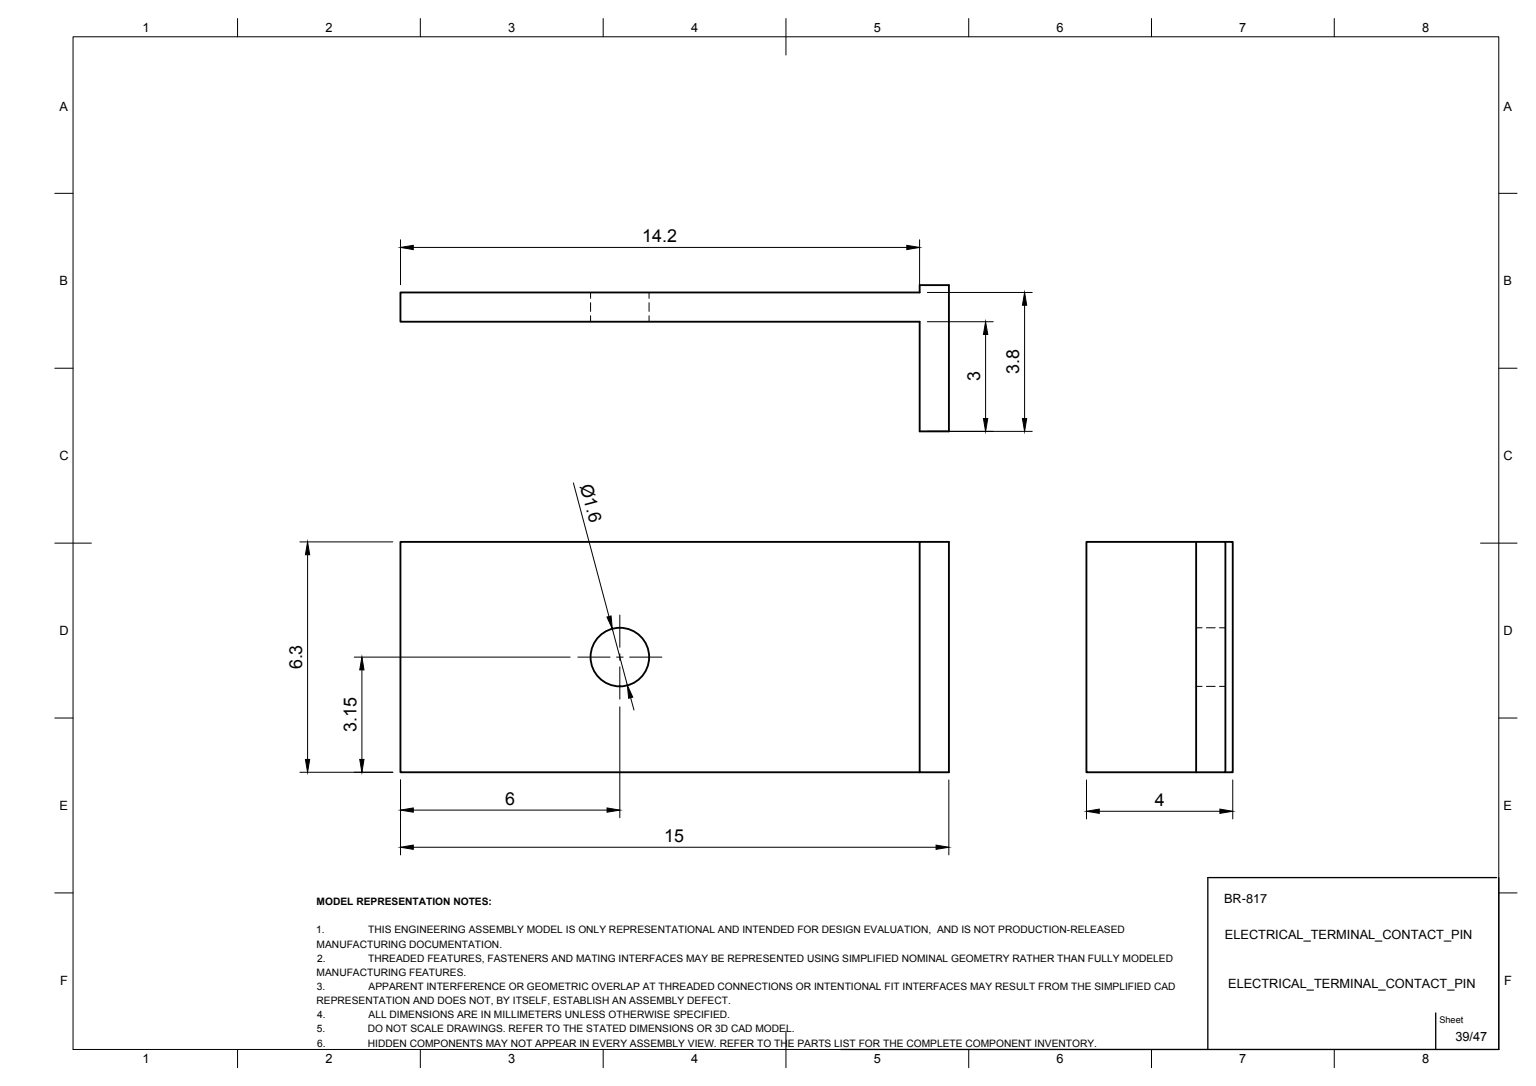
ISO-10303-21;
HEADER;
FILE_DESCRIPTION((''),'2;1');
FILE_NAME('ELECTRICAL_TERMINAL_CONTACT_PIN.step','2026-10-01T22:07:29-07:00',(''),(''),'','','');
FILE_SCHEMA (('AUTOMOTIVE_DESIGN { 1 0 10303 214 3 1 1 }'));
ENDSEC;
DATA;
#10=MECHANICAL_DESIGN_GEOMETRIC_PRESENTATION_REPRESENTATION('',(#570),#15484);
#499=SHAPE_REPRESENTATION_RELATIONSHIP('SRR','None',#15650,#534) ;
#534=ADVANCED_BREP_SHAPE_REPRESENTATION('',(#611),#15474) ;
#570=STYLED_ITEM('',(#15834),#611) ;
#611=MANIFOLD_SOLID_BREP('ELECTRICAL_TERMINAL_CONTACT_PIN',#8281) ;
#793=CYLINDRICAL_SURFACE('',#9781,0.08) ;
#876=FACE_BOUND('',#2357,.T.) ;
#877=FACE_BOUND('',#2360,.T.) ;
#1325=CIRCLE('',#9782,0.08) ;
#1326=CIRCLE('',#9783,0.08) ;
#1789=FACE_OUTER_BOUND('',#2355,.T.) ;
#1790=FACE_OUTER_BOUND('',#2356,.T.) ;
#1791=FACE_OUTER_BOUND('',#2358,.T.) ;
#1792=FACE_OUTER_BOUND('',#2359,.T.) ;
#1793=FACE_OUTER_BOUND('',#2361,.T.) ;
#1794=FACE_OUTER_BOUND('',#2362,.T.) ;
#1795=FACE_OUTER_BOUND('',#2363,.T.) ;
#1796=FACE_OUTER_BOUND('',#2364,.T.) ;
#1797=FACE_OUTER_BOUND('',#2365,.T.) ;
#1798=FACE_OUTER_BOUND('',#2366,.T.) ;
#1799=FACE_OUTER_BOUND('',#2367,.T.) ;
#2355=EDGE_LOOP('',(#7269,#7270,#7271,#7272)) ;
#2356=EDGE_LOOP('',(#7273,#7274,#7275,#7276)) ;
#2357=EDGE_LOOP('',(#7277)) ;
#2358=EDGE_LOOP('',(#7278,#7279,#7280,#7281)) ;
#2359=EDGE_LOOP('',(#7282,#7283,#7284,#7285)) ;
#2360=EDGE_LOOP('',(#7286)) ;
#2361=EDGE_LOOP('',(#7287,#7288,#7289,#7290)) ;
#2362=EDGE_LOOP('',(#7291,#7292,#7293,#7294)) ;
#2363=EDGE_LOOP('',(#7295,#7296,#7297,#7298)) ;
#2364=EDGE_LOOP('',(#7299,#7300,#7301,#7302,#7303,#7304,#7305,#7306)) ;
#2365=EDGE_LOOP('',(#7307,#7308,#7309,#7310)) ;
#2366=EDGE_LOOP('',(#7311,#7312,#7313,#7314,#7315,#7316,#7317,#7318)) ;
#2367=EDGE_LOOP('',(#7319,#7320,#7321,#7322)) ;
#2820=LINE('',#15076,#3294) ;
#2821=LINE('',#15081,#3295) ;
#2822=LINE('',#15083,#3296) ;
#2823=LINE('',#15085,#3297) ;
#2824=LINE('',#15086,#3298) ;
#2825=LINE('',#15090,#3299) ;
#2826=LINE('',#15091,#3300) ;
#2827=LINE('',#15092,#3301) ;
#2828=LINE('',#15096,#3302) ;
#2829=LINE('',#15097,#3303) ;
#2830=LINE('',#15098,#3304) ;
#2831=LINE('',#15102,#3305) ;
#2832=LINE('',#15104,#3306) ;
#2833=LINE('',#15106,#3307) ;
#2834=LINE('',#15107,#3308) ;
#2835=LINE('',#15110,#3309) ;
#2836=LINE('',#15112,#3310) ;
#2837=LINE('',#15113,#3311) ;
#2838=LINE('',#15116,#3312) ;
#2839=LINE('',#15118,#3313) ;
#2840=LINE('',#15119,#3314) ;
#2841=LINE('',#15121,#3315) ;
#2842=LINE('',#15122,#3316) ;
#2843=LINE('',#15124,#3317) ;
#2844=LINE('',#15126,#3318) ;
#3294=VECTOR('',#12507,0.08) ;
#3295=VECTOR('',#12512,1.) ;
#3296=VECTOR('',#12513,1.) ;
#3297=VECTOR('',#12514,1.) ;
#3298=VECTOR('',#12515,1.) ;
#3299=VECTOR('',#12518,1.) ;
#3300=VECTOR('',#12519,1.) ;
#3301=VECTOR('',#12520,1.) ;
#3302=VECTOR('',#12523,1.) ;
#3303=VECTOR('',#12524,1.) ;
#3304=VECTOR('',#12525,1.) ;
#3305=VECTOR('',#12528,1.) ;
#3306=VECTOR('',#12529,1.) ;
#3307=VECTOR('',#12530,1.) ;
#3308=VECTOR('',#12531,1.) ;
#3309=VECTOR('',#12534,1.) ;
#3310=VECTOR('',#12535,1.) ;
#3311=VECTOR('',#12536,1.) ;
#3312=VECTOR('',#12539,1.) ;
#3313=VECTOR('',#12540,1.) ;
#3314=VECTOR('',#12541,1.) ;
#3315=VECTOR('',#12544,1.) ;
#3316=VECTOR('',#12545,1.) ;
#3317=VECTOR('',#12548,1.) ;
#3318=VECTOR('',#12551,1.) ;
#4052=VERTEX_POINT('',#15073) ;
#4053=VERTEX_POINT('',#15075) ;
#4054=VERTEX_POINT('',#15079) ;
#4055=VERTEX_POINT('',#15080) ;
#4056=VERTEX_POINT('',#15082) ;
#4057=VERTEX_POINT('',#15084) ;
#4058=VERTEX_POINT('',#15088) ;
#4059=VERTEX_POINT('',#15089) ;
#4060=VERTEX_POINT('',#15094) ;
#4061=VERTEX_POINT('',#15095) ;
#4062=VERTEX_POINT('',#15100) ;
#4063=VERTEX_POINT('',#15101) ;
#4064=VERTEX_POINT('',#15103) ;
#4065=VERTEX_POINT('',#15105) ;
#4066=VERTEX_POINT('',#15109) ;
#4067=VERTEX_POINT('',#15111) ;
#4068=VERTEX_POINT('',#15115) ;
#4069=VERTEX_POINT('',#15117) ;
#5139=EDGE_CURVE('',#4052,#4052,#1325,.T.) ;
#5140=EDGE_CURVE('',#4052,#4053,#2820,.T.) ;
#5141=EDGE_CURVE('',#4053,#4053,#1326,.T.) ;
#5142=EDGE_CURVE('',#4054,#4055,#2821,.T.) ;
#5143=EDGE_CURVE('',#4056,#4054,#2822,.T.) ;
#5144=EDGE_CURVE('',#4057,#4056,#2823,.T.) ;
#5145=EDGE_CURVE('',#4057,#4055,#2824,.T.) ;
#5146=EDGE_CURVE('',#4058,#4059,#2825,.T.) ;
#5147=EDGE_CURVE('',#4059,#4057,#2826,.T.) ;
#5148=EDGE_CURVE('',#4056,#4058,#2827,.T.) ;
#5149=EDGE_CURVE('',#4060,#4061,#2828,.T.) ;
#5150=EDGE_CURVE('',#4059,#4060,#2829,.T.) ;
#5151=EDGE_CURVE('',#4058,#4061,#2830,.T.) ;
#5152=EDGE_CURVE('',#4062,#4063,#2831,.T.) ;
#5153=EDGE_CURVE('',#4063,#4064,#2832,.T.) ;
#5154=EDGE_CURVE('',#4064,#4065,#2833,.T.) ;
#5155=EDGE_CURVE('',#4065,#4062,#2834,.T.) ;
#5156=EDGE_CURVE('',#4061,#4066,#2835,.T.) ;
#5157=EDGE_CURVE('',#4066,#4067,#2836,.T.) ;
#5158=EDGE_CURVE('',#4067,#4060,#2837,.T.) ;
#5159=EDGE_CURVE('',#4055,#4068,#2838,.T.) ;
#5160=EDGE_CURVE('',#4068,#4069,#2839,.T.) ;
#5161=EDGE_CURVE('',#4069,#4054,#2840,.T.) ;
#5162=EDGE_CURVE('',#4066,#4064,#2841,.T.) ;
#5163=EDGE_CURVE('',#4069,#4065,#2842,.T.) ;
#5164=EDGE_CURVE('',#4068,#4062,#2843,.T.) ;
#5165=EDGE_CURVE('',#4067,#4063,#2844,.T.) ;
#7269=ORIENTED_EDGE('',*,*,#5139,.F.) ;
#7270=ORIENTED_EDGE('',*,*,#5140,.T.) ;
#7271=ORIENTED_EDGE('',*,*,#5141,.F.) ;
#7272=ORIENTED_EDGE('',*,*,#5140,.F.) ;
#7273=ORIENTED_EDGE('',*,*,#5142,.F.) ;
#7274=ORIENTED_EDGE('',*,*,#5143,.F.) ;
#7275=ORIENTED_EDGE('',*,*,#5144,.F.) ;
#7276=ORIENTED_EDGE('',*,*,#5145,.T.) ;
#7277=ORIENTED_EDGE('',*,*,#5139,.T.) ;
#7278=ORIENTED_EDGE('',*,*,#5146,.T.) ;
#7279=ORIENTED_EDGE('',*,*,#5147,.T.) ;
#7280=ORIENTED_EDGE('',*,*,#5144,.T.) ;
#7281=ORIENTED_EDGE('',*,*,#5148,.T.) ;
#7282=ORIENTED_EDGE('',*,*,#5149,.F.) ;
#7283=ORIENTED_EDGE('',*,*,#5150,.F.) ;
#7284=ORIENTED_EDGE('',*,*,#5146,.F.) ;
#7285=ORIENTED_EDGE('',*,*,#5151,.T.) ;
#7286=ORIENTED_EDGE('',*,*,#5141,.T.) ;
#7287=ORIENTED_EDGE('',*,*,#5152,.T.) ;
#7288=ORIENTED_EDGE('',*,*,#5153,.T.) ;
#7289=ORIENTED_EDGE('',*,*,#5154,.T.) ;
#7290=ORIENTED_EDGE('',*,*,#5155,.T.) ;
#7291=ORIENTED_EDGE('',*,*,#5149,.T.) ;
#7292=ORIENTED_EDGE('',*,*,#5156,.T.) ;
#7293=ORIENTED_EDGE('',*,*,#5157,.T.) ;
#7294=ORIENTED_EDGE('',*,*,#5158,.T.) ;
#7295=ORIENTED_EDGE('',*,*,#5142,.T.) ;
#7296=ORIENTED_EDGE('',*,*,#5159,.T.) ;
#7297=ORIENTED_EDGE('',*,*,#5160,.T.) ;
#7298=ORIENTED_EDGE('',*,*,#5161,.T.) ;
#7299=ORIENTED_EDGE('',*,*,#5154,.F.) ;
#7300=ORIENTED_EDGE('',*,*,#5162,.F.) ;
#7301=ORIENTED_EDGE('',*,*,#5156,.F.) ;
#7302=ORIENTED_EDGE('',*,*,#5151,.F.) ;
#7303=ORIENTED_EDGE('',*,*,#5148,.F.) ;
#7304=ORIENTED_EDGE('',*,*,#5143,.T.) ;
#7305=ORIENTED_EDGE('',*,*,#5161,.F.) ;
#7306=ORIENTED_EDGE('',*,*,#5163,.T.) ;
#7307=ORIENTED_EDGE('',*,*,#5164,.T.) ;
#7308=ORIENTED_EDGE('',*,*,#5155,.F.) ;
#7309=ORIENTED_EDGE('',*,*,#5163,.F.) ;
#7310=ORIENTED_EDGE('',*,*,#5160,.F.) ;
#7311=ORIENTED_EDGE('',*,*,#5152,.F.) ;
#7312=ORIENTED_EDGE('',*,*,#5164,.F.) ;
#7313=ORIENTED_EDGE('',*,*,#5159,.F.) ;
#7314=ORIENTED_EDGE('',*,*,#5145,.F.) ;
#7315=ORIENTED_EDGE('',*,*,#5147,.F.) ;
#7316=ORIENTED_EDGE('',*,*,#5150,.T.) ;
#7317=ORIENTED_EDGE('',*,*,#5158,.F.) ;
#7318=ORIENTED_EDGE('',*,*,#5165,.T.) ;
#7319=ORIENTED_EDGE('',*,*,#5162,.T.) ;
#7320=ORIENTED_EDGE('',*,*,#5153,.F.) ;
#7321=ORIENTED_EDGE('',*,*,#5165,.F.) ;
#7322=ORIENTED_EDGE('',*,*,#5157,.F.) ;
#7695=PLANE('',#9784) ;
#7696=PLANE('',#9785) ;
#7697=PLANE('',#9786) ;
#7698=PLANE('',#9787) ;
#7699=PLANE('',#9788) ;
#7700=PLANE('',#9789) ;
#7701=PLANE('',#9790) ;
#7702=PLANE('',#9791) ;
#7703=PLANE('',#9792) ;
#7704=PLANE('',#9793) ;
#8176=ADVANCED_FACE('',(#1789),#793,.F.) ;
#8177=ADVANCED_FACE('',(#1790,#876),#7695,.F.) ;
#8178=ADVANCED_FACE('',(#1791),#7696,.T.) ;
#8179=ADVANCED_FACE('',(#1792,#877),#7697,.F.) ;
#8180=ADVANCED_FACE('',(#1793),#7698,.F.) ;
#8181=ADVANCED_FACE('',(#1794),#7699,.T.) ;
#8182=ADVANCED_FACE('',(#1795),#7700,.T.) ;
#8183=ADVANCED_FACE('',(#1796),#7701,.F.) ;
#8184=ADVANCED_FACE('',(#1797),#7702,.F.) ;
#8185=ADVANCED_FACE('',(#1798),#7703,.F.) ;
#8186=ADVANCED_FACE('',(#1799),#7704,.F.) ;
#8281=CLOSED_SHELL('',(#8176,#8177,#8178,#8179,#8180,#8181,#8182,#8183,
#8184,#8185,#8186)) ;
#9780=AXIS2_PLACEMENT_3D('',#15071,#12501,#12502) ;
#9781=AXIS2_PLACEMENT_3D('',#15072,#12503,#12504) ;
#9782=AXIS2_PLACEMENT_3D('',#15074,#12505,#12506) ;
#9783=AXIS2_PLACEMENT_3D('',#15077,#12508,#12509) ;
#9784=AXIS2_PLACEMENT_3D('',#15078,#12510,#12511) ;
#9785=AXIS2_PLACEMENT_3D('',#15087,#12516,#12517) ;
#9786=AXIS2_PLACEMENT_3D('',#15093,#12521,#12522) ;
#9787=AXIS2_PLACEMENT_3D('',#15099,#12526,#12527) ;
#9788=AXIS2_PLACEMENT_3D('',#15108,#12532,#12533) ;
#9789=AXIS2_PLACEMENT_3D('',#15114,#12537,#12538) ;
#9790=AXIS2_PLACEMENT_3D('',#15120,#12542,#12543) ;
#9791=AXIS2_PLACEMENT_3D('',#15123,#12546,#12547) ;
#9792=AXIS2_PLACEMENT_3D('',#15125,#12549,#12550) ;
#9793=AXIS2_PLACEMENT_3D('',#15127,#12552,#12553) ;
#12501=DIRECTION('axis',(0.,0.,1.)) ;
#12502=DIRECTION('refdir',(1.,0.,0.)) ;
#12503=DIRECTION('center_axis',(1.,0.,0.)) ;
#12504=DIRECTION('ref_axis',(0.,0.,-1.)) ;
#12505=DIRECTION('center_axis',(1.,0.,0.)) ;
#12506=DIRECTION('ref_axis',(0.,0.,-1.)) ;
#12507=DIRECTION('',(1.,0.,0.)) ;
#12508=DIRECTION('center_axis',(-1.,0.,0.)) ;
#12509=DIRECTION('ref_axis',(0.,0.,-1.)) ;
#12510=DIRECTION('center_axis',(1.,0.,0.)) ;
#12511=DIRECTION('ref_axis',(0.,0.,-1.)) ;
#12512=DIRECTION('',(0.,1.,0.)) ;
#12513=DIRECTION('',(0.,0.,-1.)) ;
#12514=DIRECTION('',(0.,-1.,0.)) ;
#12515=DIRECTION('',(0.,0.,-1.)) ;
#12516=DIRECTION('center_axis',(0.,0.,1.)) ;
#12517=DIRECTION('ref_axis',(1.,0.,0.)) ;
#12518=DIRECTION('',(0.,1.,0.)) ;
#12519=DIRECTION('',(-1.,0.,0.)) ;
#12520=DIRECTION('',(1.,0.,0.)) ;
#12521=DIRECTION('center_axis',(-1.,0.,0.)) ;
#12522=DIRECTION('ref_axis',(0.,0.,1.)) ;
#12523=DIRECTION('',(0.,-1.,0.)) ;
#12524=DIRECTION('',(0.,0.,-1.)) ;
#12525=DIRECTION('',(0.,0.,-1.)) ;
#12526=DIRECTION('center_axis',(0.,0.,1.)) ;
#12527=DIRECTION('ref_axis',(1.,0.,0.)) ;
#12528=DIRECTION('',(1.,0.,0.)) ;
#12529=DIRECTION('',(0.,-1.,0.)) ;
#12530=DIRECTION('',(-1.,0.,0.)) ;
#12531=DIRECTION('',(0.,1.,0.)) ;
#12532=DIRECTION('center_axis',(0.,0.,1.)) ;
#12533=DIRECTION('ref_axis',(1.,0.,0.)) ;
#12534=DIRECTION('',(1.,0.,0.)) ;
#12535=DIRECTION('',(0.,1.,0.)) ;
#12536=DIRECTION('',(-1.,0.,0.)) ;
#12537=DIRECTION('center_axis',(0.,0.,1.)) ;
#12538=DIRECTION('ref_axis',(1.,0.,0.)) ;
#12539=DIRECTION('',(-1.,0.,0.)) ;
#12540=DIRECTION('',(0.,-1.,0.)) ;
#12541=DIRECTION('',(1.,0.,0.)) ;
#12542=DIRECTION('center_axis',(0.,1.,0.)) ;
#12543=DIRECTION('ref_axis',(0.,0.,1.)) ;
#12544=DIRECTION('',(0.,0.,-1.)) ;
#12545=DIRECTION('',(0.,0.,-1.)) ;
#12546=DIRECTION('center_axis',(1.,0.,0.)) ;
#12547=DIRECTION('ref_axis',(0.,0.,-1.)) ;
#12548=DIRECTION('',(0.,0.,-1.)) ;
#12549=DIRECTION('center_axis',(0.,-1.,0.)) ;
#12550=DIRECTION('ref_axis',(0.,0.,-1.)) ;
#12551=DIRECTION('',(0.,0.,-1.)) ;
#12552=DIRECTION('center_axis',(-1.,0.,0.)) ;
#12553=DIRECTION('ref_axis',(0.,0.,1.)) ;
#15071=CARTESIAN_POINT('',(0.,0.,0.)) ;
#15072=CARTESIAN_POINT('Origin',(3.65,0.,1.2)) ;
#15073=CARTESIAN_POINT('',(3.6,-9.79717439317883E-18,1.28)) ;
#15074=CARTESIAN_POINT('Origin',(3.6,0.,1.2)) ;
#15075=CARTESIAN_POINT('',(3.68,9.79717439317883E-18,1.28)) ;
#15076=CARTESIAN_POINT('',(3.65,-9.79717439317883E-18,1.28)) ;
#15077=CARTESIAN_POINT('Origin',(3.68,0.,1.2)) ;
#15078=CARTESIAN_POINT('Origin',(3.6,0.,1.05)) ;
#15079=CARTESIAN_POINT('',(3.6,-0.315,0.38)) ;
#15080=CARTESIAN_POINT('',(3.6,0.315,0.38)) ;
#15081=CARTESIAN_POINT('',(3.6,0.,0.38)) ;
#15082=CARTESIAN_POINT('',(3.6,-0.315,1.8)) ;
#15083=CARTESIAN_POINT('',(3.6,-0.315,1.05)) ;
#15084=CARTESIAN_POINT('',(3.6,0.315,1.8)) ;
#15085=CARTESIAN_POINT('',(3.6,0.,1.8)) ;
#15086=CARTESIAN_POINT('',(3.6,0.315,1.05)) ;
#15087=CARTESIAN_POINT('Origin',(3.64,0.,1.8)) ;
#15088=CARTESIAN_POINT('',(3.68,-0.315,1.8)) ;
#15089=CARTESIAN_POINT('',(3.68,0.315,1.8)) ;
#15090=CARTESIAN_POINT('',(3.68,0.,1.8)) ;
#15091=CARTESIAN_POINT('',(3.64,0.315,1.8)) ;
#15092=CARTESIAN_POINT('',(3.64,-0.315,1.8)) ;
#15093=CARTESIAN_POINT('Origin',(3.68,0.,1.05)) ;
#15094=CARTESIAN_POINT('',(3.68,0.315,0.38)) ;
#15095=CARTESIAN_POINT('',(3.68,-0.315,0.38)) ;
#15096=CARTESIAN_POINT('',(3.68,0.,0.38)) ;
#15097=CARTESIAN_POINT('',(3.68,0.315,1.05)) ;
#15098=CARTESIAN_POINT('',(3.68,-0.315,1.05)) ;
#15099=CARTESIAN_POINT('Origin',(3.5,0.,0.3)) ;
#15100=CARTESIAN_POINT('',(3.3,0.315,0.3)) ;
#15101=CARTESIAN_POINT('',(3.7,0.315,0.3)) ;
#15102=CARTESIAN_POINT('',(3.5,0.315,0.3)) ;
#15103=CARTESIAN_POINT('',(3.7,-0.315,0.3)) ;
#15104=CARTESIAN_POINT('',(3.7,0.,0.3)) ;
#15105=CARTESIAN_POINT('',(3.3,-0.315,0.3)) ;
#15106=CARTESIAN_POINT('',(3.5,-0.315,0.3)) ;
#15107=CARTESIAN_POINT('',(3.3,0.,0.3)) ;
#15108=CARTESIAN_POINT('Origin',(3.5,0.,0.38)) ;
#15109=CARTESIAN_POINT('',(3.7,-0.315,0.38)) ;
#15110=CARTESIAN_POINT('',(3.5,-0.315,0.38)) ;
#15111=CARTESIAN_POINT('',(3.7,0.315,0.38)) ;
#15112=CARTESIAN_POINT('',(3.7,0.,0.38)) ;
#15113=CARTESIAN_POINT('',(3.5,0.315,0.38)) ;
#15114=CARTESIAN_POINT('Origin',(3.5,0.,0.38)) ;
#15115=CARTESIAN_POINT('',(3.3,0.315,0.38)) ;
#15116=CARTESIAN_POINT('',(3.5,0.315,0.38)) ;
#15117=CARTESIAN_POINT('',(3.3,-0.315,0.38)) ;
#15118=CARTESIAN_POINT('',(3.3,0.,0.38)) ;
#15119=CARTESIAN_POINT('',(3.5,-0.315,0.38)) ;
#15120=CARTESIAN_POINT('Origin',(3.5,-0.315,0.34)) ;
#15121=CARTESIAN_POINT('',(3.7,-0.315,0.34)) ;
#15122=CARTESIAN_POINT('',(3.3,-0.315,0.34)) ;
#15123=CARTESIAN_POINT('Origin',(3.3,0.,0.34)) ;
#15124=CARTESIAN_POINT('',(3.3,0.315,0.34)) ;
#15125=CARTESIAN_POINT('Origin',(3.5,0.315,0.34)) ;
#15126=CARTESIAN_POINT('',(3.7,0.315,0.34)) ;
#15127=CARTESIAN_POINT('Origin',(3.7,0.,0.34)) ;
#15431=UNCERTAINTY_MEASURE_WITH_UNIT(LENGTH_MEASURE(0.001),#15485,
'DISTANCE_ACCURACY_VALUE',
'Maximum model space distance between geometric entities at asserted c
onnectivities') ;
#15441=UNCERTAINTY_MEASURE_WITH_UNIT(LENGTH_MEASURE(0.001),#15485,
'DISTANCE_ACCURACY_VALUE',
'Maximum model space distance between geometric entities at asserted c
onnectivities') ;
#15474=(
GEOMETRIC_REPRESENTATION_CONTEXT(3)
GLOBAL_UNCERTAINTY_ASSIGNED_CONTEXT((#15431))
GLOBAL_UNIT_ASSIGNED_CONTEXT((#15485,#15487,#15488))
REPRESENTATION_CONTEXT('','3D')
) ;
#15484=(
GEOMETRIC_REPRESENTATION_CONTEXT(3)
GLOBAL_UNCERTAINTY_ASSIGNED_CONTEXT((#15441))
GLOBAL_UNIT_ASSIGNED_CONTEXT((#15485,#15487,#15488))
REPRESENTATION_CONTEXT('','3D')
) ;
#15485=(
LENGTH_UNIT()
NAMED_UNIT(*)
SI_UNIT(.CENTI.,.METRE.)
) ;
#15487=(
NAMED_UNIT(*)
PLANE_ANGLE_UNIT()
SI_UNIT($,.RADIAN.)
) ;
#15488=(
NAMED_UNIT(*)
SI_UNIT($,.STERADIAN.)
SOLID_ANGLE_UNIT()
) ;
#15521=SHAPE_DEFINITION_REPRESENTATION(#15589,#15650) ;
#15589=PRODUCT_DEFINITION_SHAPE('',$,#15693) ;
#15650=SHAPE_REPRESENTATION('',(#9780),#15474) ;
#15660=PRODUCT_DEFINITION_CONTEXT('part definition',#15788,'design') ;
#15693=PRODUCT_DEFINITION('ELECTRICAL_TERMINAL_CONTACT_PIN',
'ELECTRICAL_TERMINAL_CONTACT_PIN',#15735,#15660) ;
#15735=PRODUCT_DEFINITION_FORMATION('',$,#15822) ;
#15788=APPLICATION_CONTEXT(
'Core Data for Automotive Mechanical Design Process') ;
#15789=PRODUCT_CONTEXT('part definition',#15788,'mechanical') ;
#15822=PRODUCT('ELECTRICAL_TERMINAL_CONTACT_PIN',
'ELECTRICAL_TERMINAL_CONTACT_PIN',$,(#15789)) ;
#15834=PRESENTATION_STYLE_ASSIGNMENT((#15846)) ;
#15846=SURFACE_STYLE_USAGE(.BOTH.,#15858) ;
#15858=SURFACE_SIDE_STYLE('',(#15870)) ;
#15870=SURFACE_STYLE_FILL_AREA(#15882) ;
#15882=FILL_AREA_STYLE('Brass - Polished',(#15894)) ;
#15894=FILL_AREA_STYLE_COLOUR('Brass - Polished',#15906) ;
#15906=COLOUR_RGB('Brass - Polished', 0.08235294, 0.09019608, 0.10196078) ;
ENDSEC;
END-ISO-10303-21;
